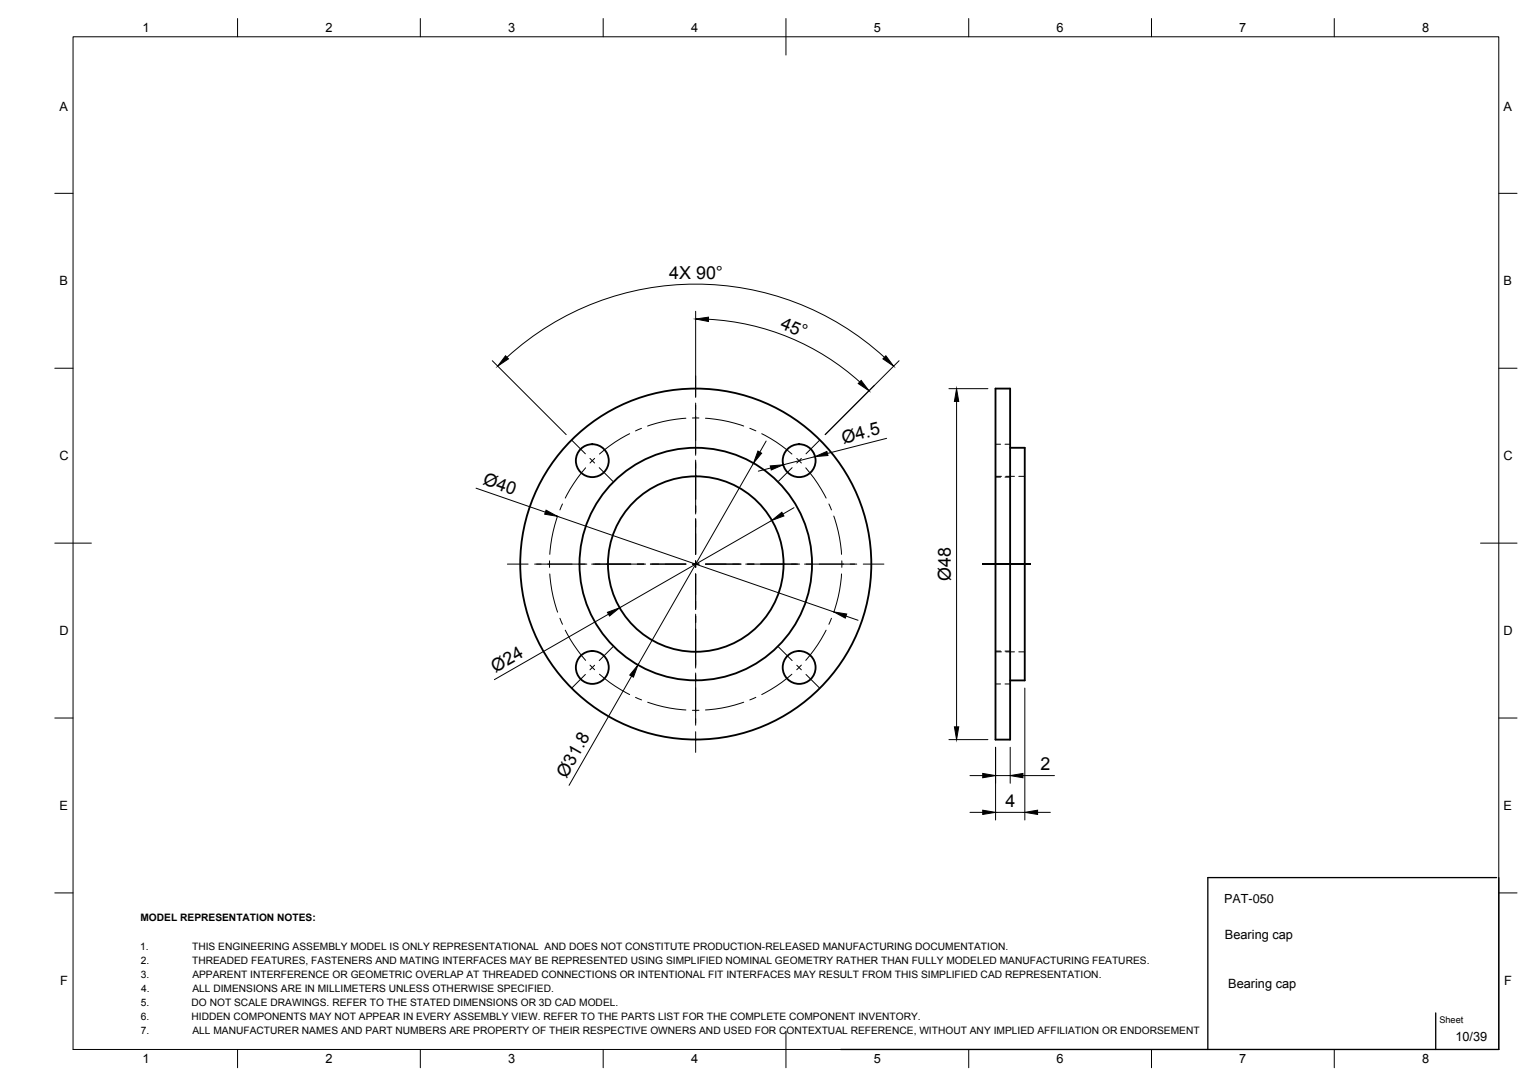
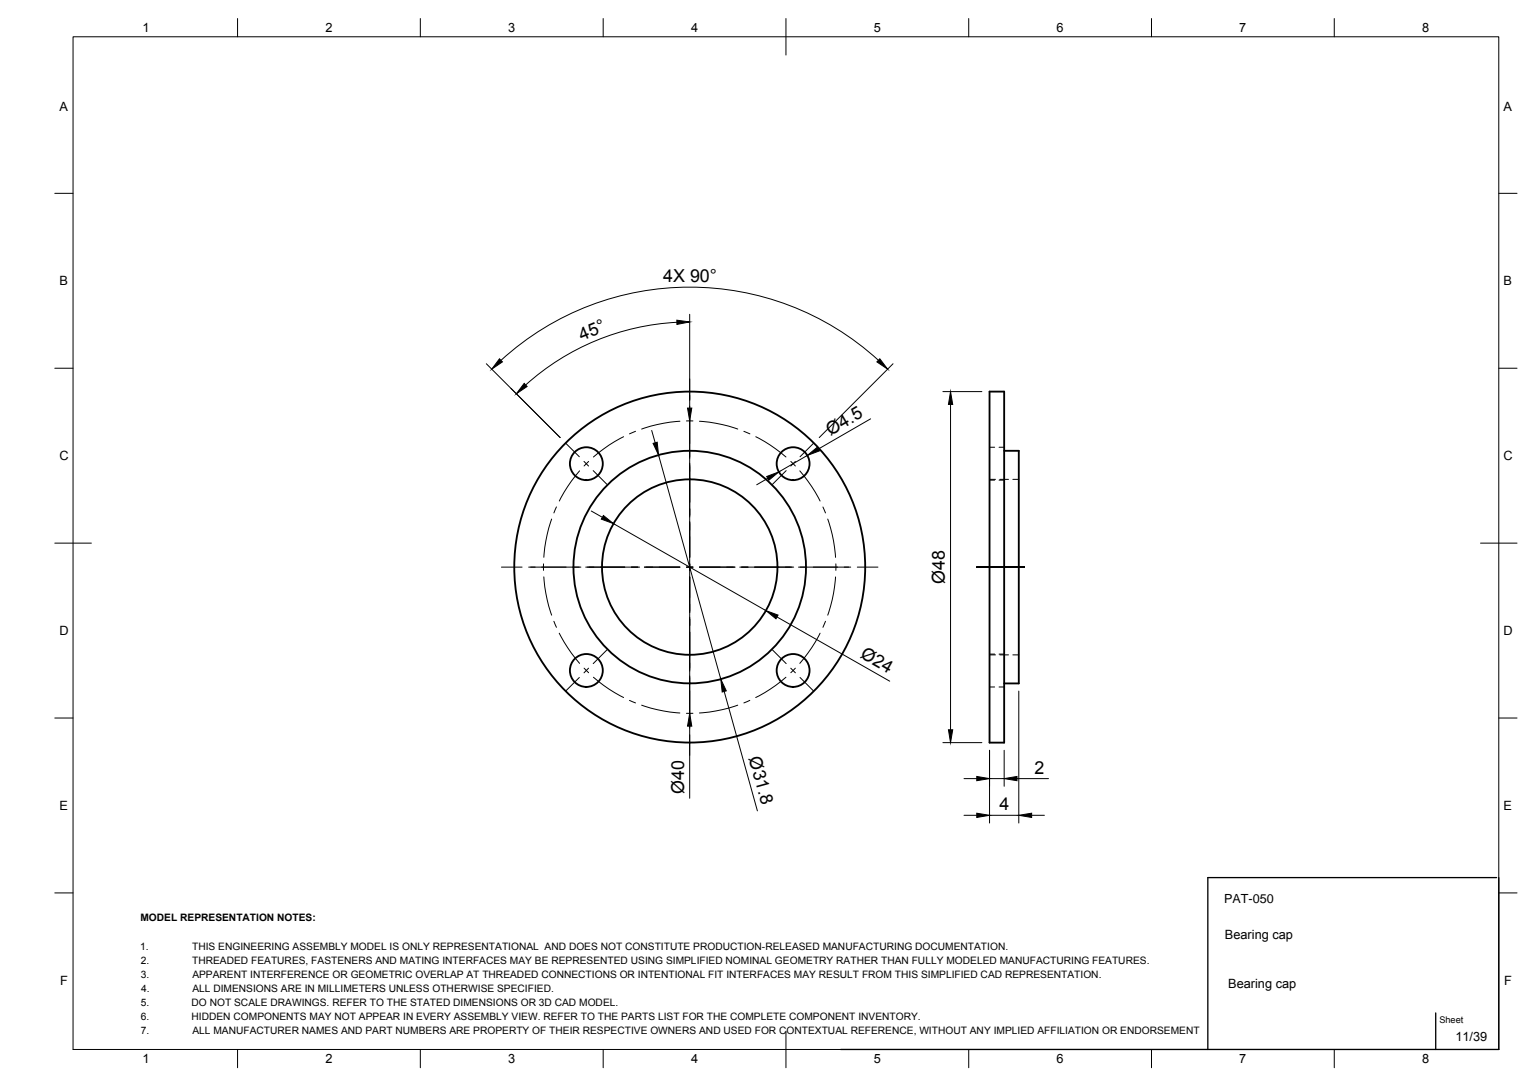
ISO-10303-21;
HEADER;
/* Generated by software containing ST-Developer
 * from STEP Tools, Inc. (www.steptools.com) 
 */

FILE_DESCRIPTION(
/* description */ ('Hand wheel with handle and shaft collar'),
/* implementation_level */ '2;1');

FILE_NAME(
/* name */ 'Bearing cap.step',
/* time_stamp */ '2026-10-28T03:23:19-07:00',
/* author */ (''),
/* organization */ (''),
/* preprocessor_version */ 'ST-DEVELOPER v20.2',
/* originating_system */ 'Autodesk Translation Framework v15.17.0.0',
/* authorisation */ '');

FILE_SCHEMA (('AUTOMOTIVE_DESIGN { 1 0 10303 214 3 1 1 }'));
ENDSEC;

DATA;
#10=MECHANICAL_DESIGN_GEOMETRIC_PRESENTATION_REPRESENTATION('',(#400),#10510);
#336=SHAPE_REPRESENTATION_RELATIONSHIP('SRR','None',#10652,#368);
#368=ADVANCED_BREP_SHAPE_REPRESENTATION('',(#447),#10479);
#400=STYLED_ITEM('',(#10908),#447);
#447=MANIFOLD_SOLID_BREP('Body1',#5299);
#514=FACE_BOUND('',#1161,.T.);
#515=FACE_BOUND('',#1165,.T.);
#516=FACE_BOUND('',#1166,.T.);
#517=FACE_BOUND('',#1167,.T.);
#518=FACE_BOUND('',#1168,.T.);
#519=FACE_BOUND('',#1169,.T.);
#520=FACE_BOUND('',#1171,.T.);
#521=FACE_BOUND('',#1172,.T.);
#522=FACE_BOUND('',#1173,.T.);
#523=FACE_BOUND('',#1174,.T.);
#524=FACE_BOUND('',#1175,.T.);
#628=PLANE('',#5795);
#629=PLANE('',#5802);
#630=PLANE('',#5803);
#808=FACE_OUTER_BOUND('',#1155,.T.);
#809=FACE_OUTER_BOUND('',#1156,.T.);
#810=FACE_OUTER_BOUND('',#1157,.T.);
#811=FACE_OUTER_BOUND('',#1158,.T.);
#812=FACE_OUTER_BOUND('',#1159,.T.);
#813=FACE_OUTER_BOUND('',#1160,.T.);
#814=FACE_OUTER_BOUND('',#1162,.T.);
#815=FACE_OUTER_BOUND('',#1163,.T.);
#816=FACE_OUTER_BOUND('',#1164,.T.);
#817=FACE_OUTER_BOUND('',#1170,.T.);
#1155=EDGE_LOOP('',(#3767,#3768,#3769,#3770));
#1156=EDGE_LOOP('',(#3771,#3772,#3773,#3774));
#1157=EDGE_LOOP('',(#3775,#3776,#3777,#3778));
#1158=EDGE_LOOP('',(#3779,#3780,#3781,#3782));
#1159=EDGE_LOOP('',(#3783,#3784,#3785,#3786));
#1160=EDGE_LOOP('',(#3787));
#1161=EDGE_LOOP('',(#3788));
#1162=EDGE_LOOP('',(#3789,#3790,#3791,#3792));
#1163=EDGE_LOOP('',(#3793,#3794,#3795,#3796));
#1164=EDGE_LOOP('',(#3797));
#1165=EDGE_LOOP('',(#3798));
#1166=EDGE_LOOP('',(#3799));
#1167=EDGE_LOOP('',(#3800));
#1168=EDGE_LOOP('',(#3801));
#1169=EDGE_LOOP('',(#3802));
#1170=EDGE_LOOP('',(#3803));
#1171=EDGE_LOOP('',(#3804));
#1172=EDGE_LOOP('',(#3805));
#1173=EDGE_LOOP('',(#3806));
#1174=EDGE_LOOP('',(#3807));
#1175=EDGE_LOOP('',(#3808));
#1588=LINE('',#8405,#1898);
#1589=LINE('',#8411,#1899);
#1590=LINE('',#8417,#1900);
#1591=LINE('',#8423,#1901);
#1592=LINE('',#8429,#1902);
#1593=LINE('',#8436,#1903);
#1594=LINE('',#8442,#1904);
#1898=VECTOR('',#6664,0.225);
#1899=VECTOR('',#6671,0.225);
#1900=VECTOR('',#6678,0.225);
#1901=VECTOR('',#6685,0.225);
#1902=VECTOR('',#6692,1.59);
#1903=VECTOR('',#6701,1.2);
#1904=VECTOR('',#6708,2.4);
#2163=CIRCLE('',#5781,0.225);
#2164=CIRCLE('',#5782,0.225);
#2165=CIRCLE('',#5784,0.225);
#2166=CIRCLE('',#5785,0.225);
#2167=CIRCLE('',#5787,0.225);
#2168=CIRCLE('',#5788,0.225);
#2169=CIRCLE('',#5790,0.225);
#2170=CIRCLE('',#5791,0.225);
#2171=CIRCLE('',#5793,1.59);
#2172=CIRCLE('',#5794,1.59);
#2173=CIRCLE('',#5796,1.2);
#2174=CIRCLE('',#5798,1.2);
#2175=CIRCLE('',#5800,2.4);
#2176=CIRCLE('',#5801,2.4);
#2514=VERTEX_POINT('',#8402);
#2515=VERTEX_POINT('',#8404);
#2516=VERTEX_POINT('',#8408);
#2517=VERTEX_POINT('',#8410);
#2518=VERTEX_POINT('',#8414);
#2519=VERTEX_POINT('',#8416);
#2520=VERTEX_POINT('',#8420);
#2521=VERTEX_POINT('',#8422);
#2522=VERTEX_POINT('',#8426);
#2523=VERTEX_POINT('',#8428);
#2524=VERTEX_POINT('',#8432);
#2525=VERTEX_POINT('',#8435);
#2526=VERTEX_POINT('',#8439);
#2527=VERTEX_POINT('',#8441);
#3001=EDGE_CURVE('',#2514,#2514,#2163,.T.);
#3002=EDGE_CURVE('',#2514,#2515,#1588,.T.);
#3003=EDGE_CURVE('',#2515,#2515,#2164,.T.);
#3004=EDGE_CURVE('',#2516,#2516,#2165,.T.);
#3005=EDGE_CURVE('',#2516,#2517,#1589,.T.);
#3006=EDGE_CURVE('',#2517,#2517,#2166,.T.);
#3007=EDGE_CURVE('',#2518,#2518,#2167,.T.);
#3008=EDGE_CURVE('',#2518,#2519,#1590,.T.);
#3009=EDGE_CURVE('',#2519,#2519,#2168,.T.);
#3010=EDGE_CURVE('',#2520,#2520,#2169,.T.);
#3011=EDGE_CURVE('',#2520,#2521,#1591,.T.);
#3012=EDGE_CURVE('',#2521,#2521,#2170,.T.);
#3013=EDGE_CURVE('',#2522,#2522,#2171,.T.);
#3014=EDGE_CURVE('',#2522,#2523,#1592,.T.);
#3015=EDGE_CURVE('',#2523,#2523,#2172,.T.);
#3016=EDGE_CURVE('',#2524,#2524,#2173,.T.);
#3017=EDGE_CURVE('',#2524,#2525,#1593,.T.);
#3018=EDGE_CURVE('',#2525,#2525,#2174,.T.);
#3019=EDGE_CURVE('',#2526,#2526,#2175,.T.);
#3020=EDGE_CURVE('',#2526,#2527,#1594,.T.);
#3021=EDGE_CURVE('',#2527,#2527,#2176,.T.);
#3767=ORIENTED_EDGE('',*,*,#3001,.F.);
#3768=ORIENTED_EDGE('',*,*,#3002,.T.);
#3769=ORIENTED_EDGE('',*,*,#3003,.F.);
#3770=ORIENTED_EDGE('',*,*,#3002,.F.);
#3771=ORIENTED_EDGE('',*,*,#3004,.F.);
#3772=ORIENTED_EDGE('',*,*,#3005,.T.);
#3773=ORIENTED_EDGE('',*,*,#3006,.F.);
#3774=ORIENTED_EDGE('',*,*,#3005,.F.);
#3775=ORIENTED_EDGE('',*,*,#3007,.F.);
#3776=ORIENTED_EDGE('',*,*,#3008,.T.);
#3777=ORIENTED_EDGE('',*,*,#3009,.F.);
#3778=ORIENTED_EDGE('',*,*,#3008,.F.);
#3779=ORIENTED_EDGE('',*,*,#3010,.F.);
#3780=ORIENTED_EDGE('',*,*,#3011,.T.);
#3781=ORIENTED_EDGE('',*,*,#3012,.F.);
#3782=ORIENTED_EDGE('',*,*,#3011,.F.);
#3783=ORIENTED_EDGE('',*,*,#3013,.F.);
#3784=ORIENTED_EDGE('',*,*,#3014,.T.);
#3785=ORIENTED_EDGE('',*,*,#3015,.F.);
#3786=ORIENTED_EDGE('',*,*,#3014,.F.);
#3787=ORIENTED_EDGE('',*,*,#3013,.T.);
#3788=ORIENTED_EDGE('',*,*,#3016,.T.);
#3789=ORIENTED_EDGE('',*,*,#3016,.F.);
#3790=ORIENTED_EDGE('',*,*,#3017,.T.);
#3791=ORIENTED_EDGE('',*,*,#3018,.T.);
#3792=ORIENTED_EDGE('',*,*,#3017,.F.);
#3793=ORIENTED_EDGE('',*,*,#3019,.F.);
#3794=ORIENTED_EDGE('',*,*,#3020,.T.);
#3795=ORIENTED_EDGE('',*,*,#3021,.T.);
#3796=ORIENTED_EDGE('',*,*,#3020,.F.);
#3797=ORIENTED_EDGE('',*,*,#3019,.T.);
#3798=ORIENTED_EDGE('',*,*,#3015,.T.);
#3799=ORIENTED_EDGE('',*,*,#3012,.T.);
#3800=ORIENTED_EDGE('',*,*,#3009,.T.);
#3801=ORIENTED_EDGE('',*,*,#3006,.T.);
#3802=ORIENTED_EDGE('',*,*,#3003,.T.);
#3803=ORIENTED_EDGE('',*,*,#3021,.F.);
#3804=ORIENTED_EDGE('',*,*,#3018,.F.);
#3805=ORIENTED_EDGE('',*,*,#3010,.T.);
#3806=ORIENTED_EDGE('',*,*,#3007,.T.);
#3807=ORIENTED_EDGE('',*,*,#3004,.T.);
#3808=ORIENTED_EDGE('',*,*,#3001,.T.);
#4894=CYLINDRICAL_SURFACE('',#5780,0.225);
#4895=CYLINDRICAL_SURFACE('',#5783,0.225);
#4896=CYLINDRICAL_SURFACE('',#5786,0.225);
#4897=CYLINDRICAL_SURFACE('',#5789,0.225);
#4898=CYLINDRICAL_SURFACE('',#5792,1.59);
#4899=CYLINDRICAL_SURFACE('',#5797,1.2);
#4900=CYLINDRICAL_SURFACE('',#5799,2.4);
#5020=ADVANCED_FACE('',(#808),#4894,.F.);
#5021=ADVANCED_FACE('',(#809),#4895,.F.);
#5022=ADVANCED_FACE('',(#810),#4896,.F.);
#5023=ADVANCED_FACE('',(#811),#4897,.F.);
#5024=ADVANCED_FACE('',(#812),#4898,.T.);
#5025=ADVANCED_FACE('',(#813,#514),#628,.T.);
#5026=ADVANCED_FACE('',(#814),#4899,.F.);
#5027=ADVANCED_FACE('',(#815),#4900,.T.);
#5028=ADVANCED_FACE('',(#816,#515,#516,#517,#518,#519),#629,.T.);
#5029=ADVANCED_FACE('',(#817,#520,#521,#522,#523,#524),#630,.F.);
#5299=CLOSED_SHELL('',(#5020,#5021,#5022,#5023,#5024,#5025,#5026,#5027,
#5028,#5029));
#5779=AXIS2_PLACEMENT_3D('',#8400,#6658,#6659);
#5780=AXIS2_PLACEMENT_3D('',#8401,#6660,#6661);
#5781=AXIS2_PLACEMENT_3D('',#8403,#6662,#6663);
#5782=AXIS2_PLACEMENT_3D('',#8406,#6665,#6666);
#5783=AXIS2_PLACEMENT_3D('',#8407,#6667,#6668);
#5784=AXIS2_PLACEMENT_3D('',#8409,#6669,#6670);
#5785=AXIS2_PLACEMENT_3D('',#8412,#6672,#6673);
#5786=AXIS2_PLACEMENT_3D('',#8413,#6674,#6675);
#5787=AXIS2_PLACEMENT_3D('',#8415,#6676,#6677);
#5788=AXIS2_PLACEMENT_3D('',#8418,#6679,#6680);
#5789=AXIS2_PLACEMENT_3D('',#8419,#6681,#6682);
#5790=AXIS2_PLACEMENT_3D('',#8421,#6683,#6684);
#5791=AXIS2_PLACEMENT_3D('',#8424,#6686,#6687);
#5792=AXIS2_PLACEMENT_3D('',#8425,#6688,#6689);
#5793=AXIS2_PLACEMENT_3D('',#8427,#6690,#6691);
#5794=AXIS2_PLACEMENT_3D('',#8430,#6693,#6694);
#5795=AXIS2_PLACEMENT_3D('',#8431,#6695,#6696);
#5796=AXIS2_PLACEMENT_3D('',#8433,#6697,#6698);
#5797=AXIS2_PLACEMENT_3D('',#8434,#6699,#6700);
#5798=AXIS2_PLACEMENT_3D('',#8437,#6702,#6703);
#5799=AXIS2_PLACEMENT_3D('',#8438,#6704,#6705);
#5800=AXIS2_PLACEMENT_3D('',#8440,#6706,#6707);
#5801=AXIS2_PLACEMENT_3D('',#8443,#6709,#6710);
#5802=AXIS2_PLACEMENT_3D('',#8444,#6711,#6712);
#5803=AXIS2_PLACEMENT_3D('',#8445,#6713,#6714);
#6658=DIRECTION('axis',(0.,0.,1.));
#6659=DIRECTION('refdir',(1.,0.,0.));
#6660=DIRECTION('center_axis',(0.,1.,0.));
#6661=DIRECTION('ref_axis',(1.,0.,0.));
#6662=DIRECTION('center_axis',(0.,1.,0.));
#6663=DIRECTION('ref_axis',(1.,0.,0.));
#6664=DIRECTION('',(0.,1.,0.));
#6665=DIRECTION('center_axis',(0.,-1.,0.));
#6666=DIRECTION('ref_axis',(1.,0.,0.));
#6667=DIRECTION('center_axis',(0.,1.,0.));
#6668=DIRECTION('ref_axis',(1.,0.,0.));
#6669=DIRECTION('center_axis',(0.,1.,0.));
#6670=DIRECTION('ref_axis',(1.,0.,0.));
#6671=DIRECTION('',(0.,1.,0.));
#6672=DIRECTION('center_axis',(0.,-1.,0.));
#6673=DIRECTION('ref_axis',(1.,0.,0.));
#6674=DIRECTION('center_axis',(0.,1.,0.));
#6675=DIRECTION('ref_axis',(1.,0.,0.));
#6676=DIRECTION('center_axis',(0.,1.,0.));
#6677=DIRECTION('ref_axis',(1.,0.,0.));
#6678=DIRECTION('',(0.,1.,0.));
#6679=DIRECTION('center_axis',(0.,-1.,0.));
#6680=DIRECTION('ref_axis',(1.,0.,0.));
#6681=DIRECTION('center_axis',(0.,1.,0.));
#6682=DIRECTION('ref_axis',(1.,0.,0.));
#6683=DIRECTION('center_axis',(0.,1.,0.));
#6684=DIRECTION('ref_axis',(1.,0.,0.));
#6685=DIRECTION('',(0.,1.,0.));
#6686=DIRECTION('center_axis',(0.,-1.,0.));
#6687=DIRECTION('ref_axis',(1.,0.,0.));
#6688=DIRECTION('center_axis',(0.,1.,0.));
#6689=DIRECTION('ref_axis',(1.,0.,0.));
#6690=DIRECTION('center_axis',(0.,1.,0.));
#6691=DIRECTION('ref_axis',(1.,0.,0.));
#6692=DIRECTION('',(0.,-1.,0.));
#6693=DIRECTION('center_axis',(0.,-1.,0.));
#6694=DIRECTION('ref_axis',(1.,0.,0.));
#6695=DIRECTION('center_axis',(0.,1.,0.));
#6696=DIRECTION('ref_axis',(1.,0.,0.));
#6697=DIRECTION('center_axis',(0.,-1.,0.));
#6698=DIRECTION('ref_axis',(1.,0.,0.));
#6699=DIRECTION('center_axis',(0.,1.,0.));
#6700=DIRECTION('ref_axis',(1.,0.,0.));
#6701=DIRECTION('',(0.,-1.,0.));
#6702=DIRECTION('center_axis',(0.,-1.,0.));
#6703=DIRECTION('ref_axis',(1.,0.,0.));
#6704=DIRECTION('center_axis',(0.,1.,0.));
#6705=DIRECTION('ref_axis',(1.,0.,0.));
#6706=DIRECTION('center_axis',(0.,1.,0.));
#6707=DIRECTION('ref_axis',(1.,0.,0.));
#6708=DIRECTION('',(0.,-1.,0.));
#6709=DIRECTION('center_axis',(0.,1.,0.));
#6710=DIRECTION('ref_axis',(1.,0.,0.));
#6711=DIRECTION('center_axis',(0.,1.,0.));
#6712=DIRECTION('ref_axis',(1.,0.,0.));
#6713=DIRECTION('center_axis',(0.,1.,0.));
#6714=DIRECTION('ref_axis',(1.,0.,0.));
#8400=CARTESIAN_POINT('',(0.,0.,0.));
#8401=CARTESIAN_POINT('Origin',(-1.4142135623731,-1.,8.5857864376269));
#8402=CARTESIAN_POINT('',(-1.6392135623731,-0.9,8.5857864376269));
#8403=CARTESIAN_POINT('Origin',(-1.4142135623731,-0.9,8.5857864376269));
#8404=CARTESIAN_POINT('',(-1.6392135623731,-0.7,8.5857864376269));
#8405=CARTESIAN_POINT('',(-1.6392135623731,-1.,8.5857864376269));
#8406=CARTESIAN_POINT('Origin',(-1.4142135623731,-0.7,8.5857864376269));
#8407=CARTESIAN_POINT('Origin',(-1.41421356237309,-1.,11.4142135623731));
#8408=CARTESIAN_POINT('',(-1.6392135623731,-0.9,11.4142135623731));
#8409=CARTESIAN_POINT('Origin',(-1.41421356237309,-0.9,11.4142135623731));
#8410=CARTESIAN_POINT('',(-1.6392135623731,-0.7,11.4142135623731));
#8411=CARTESIAN_POINT('',(-1.6392135623731,-1.,11.4142135623731));
#8412=CARTESIAN_POINT('Origin',(-1.41421356237309,-0.7,11.4142135623731));
#8413=CARTESIAN_POINT('Origin',(1.4142135623731,-1.,11.4142135623731));
#8414=CARTESIAN_POINT('',(1.1892135623731,-0.9,11.4142135623731));
#8415=CARTESIAN_POINT('Origin',(1.4142135623731,-0.9,11.4142135623731));
#8416=CARTESIAN_POINT('',(1.1892135623731,-0.7,11.4142135623731));
#8417=CARTESIAN_POINT('',(1.1892135623731,-1.,11.4142135623731));
#8418=CARTESIAN_POINT('Origin',(1.4142135623731,-0.7,11.4142135623731));
#8419=CARTESIAN_POINT('Origin',(1.41421356237309,-1.,8.5857864376269));
#8420=CARTESIAN_POINT('',(1.18921356237309,-0.9,8.5857864376269));
#8421=CARTESIAN_POINT('Origin',(1.41421356237309,-0.9,8.5857864376269));
#8422=CARTESIAN_POINT('',(1.18921356237309,-0.7,8.5857864376269));
#8423=CARTESIAN_POINT('',(1.18921356237309,-1.,8.5857864376269));
#8424=CARTESIAN_POINT('Origin',(1.41421356237309,-0.7,8.5857864376269));
#8425=CARTESIAN_POINT('Origin',(0.,-0.7,10.));
#8426=CARTESIAN_POINT('',(-1.59,-0.5,10.));
#8427=CARTESIAN_POINT('Origin',(0.,-0.5,10.));
#8428=CARTESIAN_POINT('',(-1.59,-0.7,10.));
#8429=CARTESIAN_POINT('',(-1.59,-0.7,10.));
#8430=CARTESIAN_POINT('Origin',(0.,-0.7,10.));
#8431=CARTESIAN_POINT('Origin',(0.,-0.5,10.));
#8432=CARTESIAN_POINT('',(-1.2,-0.5,10.));
#8433=CARTESIAN_POINT('Origin',(0.,-0.5,10.));
#8434=CARTESIAN_POINT('Origin',(0.,-0.9,10.));
#8435=CARTESIAN_POINT('',(-1.2,-0.9,10.));
#8436=CARTESIAN_POINT('',(-1.2,-0.9,10.));
#8437=CARTESIAN_POINT('Origin',(0.,-0.9,10.));
#8438=CARTESIAN_POINT('Origin',(0.,-0.9,10.));
#8439=CARTESIAN_POINT('',(-2.4,-0.7,10.));
#8440=CARTESIAN_POINT('Origin',(0.,-0.7,10.));
#8441=CARTESIAN_POINT('',(-2.4,-0.9,10.));
#8442=CARTESIAN_POINT('',(-2.4,-0.9,10.));
#8443=CARTESIAN_POINT('Origin',(0.,-0.9,10.));
#8444=CARTESIAN_POINT('Origin',(0.,-0.7,10.));
#8445=CARTESIAN_POINT('Origin',(0.,-0.9,10.));
#10440=UNCERTAINTY_MEASURE_WITH_UNIT(LENGTH_MEASURE(0.001),#10511,
'DISTANCE_ACCURACY_VALUE',
'Maximum model space distance between geometric entities at asserted c
onnectivities');
#10471=UNCERTAINTY_MEASURE_WITH_UNIT(LENGTH_MEASURE(0.001),#10511,
'DISTANCE_ACCURACY_VALUE',
'Maximum model space distance between geometric entities at asserted c
onnectivities');
#10479=(
GEOMETRIC_REPRESENTATION_CONTEXT(3)
GLOBAL_UNCERTAINTY_ASSIGNED_CONTEXT((#10440))
GLOBAL_UNIT_ASSIGNED_CONTEXT((#10511,#10513,#10514))
REPRESENTATION_CONTEXT('','3D')
);
#10510=(
GEOMETRIC_REPRESENTATION_CONTEXT(3)
GLOBAL_UNCERTAINTY_ASSIGNED_CONTEXT((#10471))
GLOBAL_UNIT_ASSIGNED_CONTEXT((#10511,#10513,#10514))
REPRESENTATION_CONTEXT('','3D')
);
#10511=(
LENGTH_UNIT()
NAMED_UNIT(*)
SI_UNIT(.CENTI.,.METRE.)
);
#10513=(
NAMED_UNIT(*)
PLANE_ANGLE_UNIT()
SI_UNIT($,.RADIAN.)
);
#10514=(
NAMED_UNIT(*)
SI_UNIT($,.STERADIAN.)
SOLID_ANGLE_UNIT()
);
#10522=SHAPE_DEFINITION_REPRESENTATION(#10560,#10652);
#10560=PRODUCT_DEFINITION_SHAPE('',$,#10691);
#10652=SHAPE_REPRESENTATION('',(#5779),#10479);
#10683=PRODUCT_DEFINITION_CONTEXT('part definition',#10799,'design');
#10691=PRODUCT_DEFINITION('Bearing cap','Bearing cap',#10729,#10683);
#10729=PRODUCT_DEFINITION_FORMATION('',$,#10808);
#10799=APPLICATION_CONTEXT(
'Core Data for Automotive Mechanical Design Process');
#10800=PRODUCT_CONTEXT('part definition',#10799,'mechanical');
#10808=PRODUCT('Bearing cap','Bearing cap','Bearing cap',(#10800));
#10902=COLOUR_RGB('Grey',0.48,0.52,0.57);
#10903=FILL_AREA_STYLE_COLOUR('',#10902);
#10904=FILL_AREA_STYLE('',(#10903));
#10905=SURFACE_STYLE_FILL_AREA(#10904);
#10906=SURFACE_SIDE_STYLE('',(#10905));
#10907=SURFACE_STYLE_USAGE(.BOTH.,#10906);
#10908=PRESENTATION_STYLE_ASSIGNMENT((#10907));
ENDSEC;
END-ISO-10303-21;
